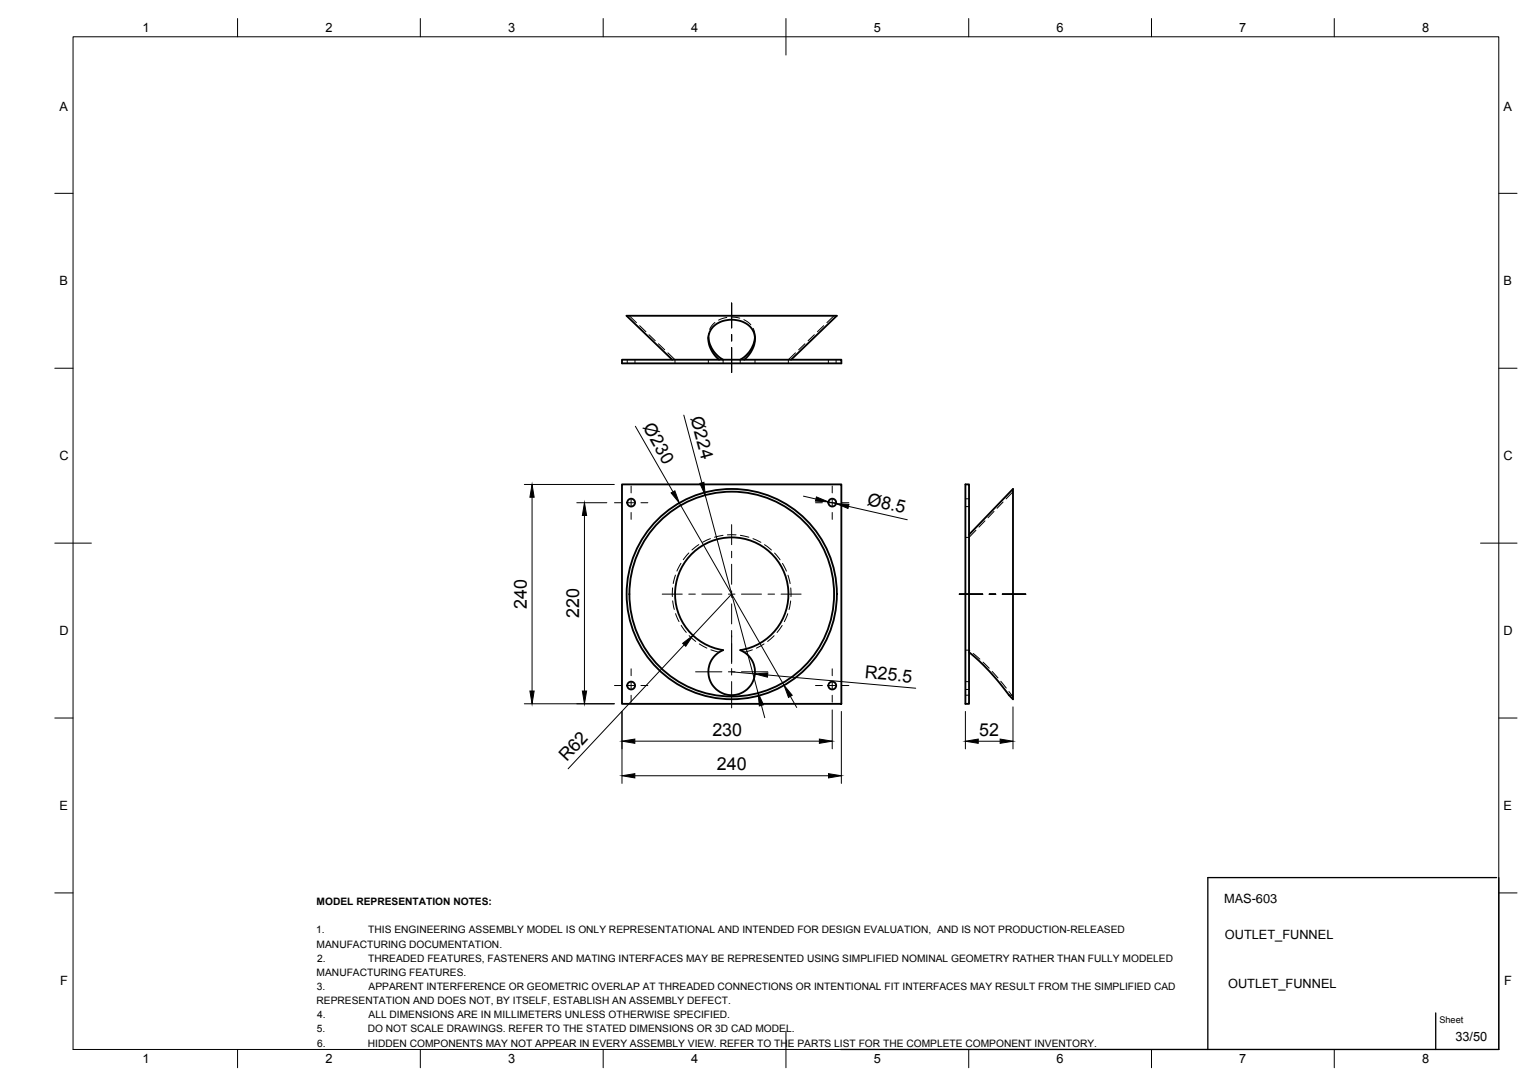
ISO-10303-21;
HEADER;
FILE_DESCRIPTION((''),'2;1');
FILE_NAME('OUTLET_FUNNEL.step','2026-10-01T22:06:14-07:00',(''),(''),'','','');
FILE_SCHEMA (('AUTOMOTIVE_DESIGN { 1 0 10303 214 3 1 1 }'));
ENDSEC;
DATA;
#10=MECHANICAL_DESIGN_GEOMETRIC_PRESENTATION_REPRESENTATION('',(#1005),#50440);
#19=B_SPLINE_CURVE_WITH_KNOTS('',3,(#46833,#46834,#46835,#46836,#46837,
#46838,#46839,#46840,#46841,#46842,#46843,#46844,#46845,#46846,#46847,#46848,
#46849,#46850,#46851,#46852,#46853,#46854,#46855,#46856,#46857,#46858,#46859,
#46860,#46861,#46862,#46863,#46864,#46865,#46866,#46867,#46868,#46869,#46870,
#46871,#46872,#46873,#46874,#46875,#46876,#46877,#46878,#46879),
 .UNSPECIFIED.,.F.,.F.,(4,2,2,2,2,2,2,2,2,2,2,2,2,2,2,2,2,2,2,3,2,2,4),
(-13.6435660379385,-13.1032156835778,-11.9806697877857,-10.8581238919937,
-10.1062638186437,-9.35440374529371,-8.60254367194372,-7.85068359859374,
-7.19512813941189,-6.53957268023004,-5.98431731311344,-5.42906194599684,
-4.87380657888023,-4.31855121176363,-3.66299575258178,-3.00744029339993,
-2.25558022004995,-1.50372014669997,-0.751860073349981,0.,1.12254589579207,
2.24509179158414,2.78544215194592),.UNSPECIFIED.) ;
#20=B_SPLINE_CURVE_WITH_KNOTS('',3,(#46883,#46884,#46885,#46886,#46887,
#46888,#46889,#46890,#46891,#46892,#46893,#46894,#46895,#46896,#46897,#46898,
#46899,#46900,#46901,#46902,#46903,#46904,#46905,#46906,#46907,#46908,#46909,
#46910,#46911,#46912,#46913,#46914,#46915,#46916,#46917,#46918,#46919,#46920,
#46921,#46922,#46923,#46924,#46925),.UNSPECIFIED.,.F.,.F.,(4,2,3,2,2,2,
2,2,2,2,2,2,2,2,2,2,2,2,2,2,4),(-2.23663632321178,-1.12254589579207,0.,
0.751860073349982,1.50372014669996,2.25558022004995,3.00744029339993,3.66299575258178,
4.31855121176363,4.87380657888023,5.42906194599683,5.98431731311343,6.53957268023004,
7.19512813941189,7.85068359859374,8.60254367194372,9.3544037452937,10.1062638186437,
10.8581238919937,11.9806697877857,13.0947602152054),.UNSPECIFIED.) ;
#913=SHAPE_REPRESENTATION_RELATIONSHIP('SRR','None',#50646,#958) ;
#958=ADVANCED_BREP_SHAPE_REPRESENTATION('',(#1060),#50415) ;
#1005=STYLED_ITEM('',(#50889),#1060) ;
#1060=MANIFOLD_SOLID_BREP('OUTLET_FUNNEL',#28672) ;
#1092=CONICAL_SURFACE('',#30829,9.,0.805803494083987) ;
#1093=CONICAL_SURFACE('',#30838,8.7,0.805803494083986) ;
#1338=FACE_BOUND('',#5137,.T.) ;
#1339=FACE_BOUND('',#5139,.T.) ;
#1340=FACE_BOUND('',#5140,.T.) ;
#1341=FACE_BOUND('',#5141,.T.) ;
#1342=FACE_BOUND('',#5142,.T.) ;
#1343=FACE_BOUND('',#5143,.T.) ;
#1344=FACE_BOUND('',#5147,.T.) ;
#1345=FACE_BOUND('',#5148,.T.) ;
#1346=FACE_BOUND('',#5149,.T.) ;
#1347=FACE_BOUND('',#5150,.T.) ;
#1348=FACE_BOUND('',#5151,.T.) ;
#1349=FACE_BOUND('',#5158,.T.) ;
#2194=PLANE('',#30824) ;
#2195=PLANE('',#30833) ;
#2196=PLANE('',#30834) ;
#2197=PLANE('',#30835) ;
#2198=PLANE('',#30836) ;
#2199=PLANE('',#30837) ;
#2200=PLANE('',#30840) ;
#3352=FACE_OUTER_BOUND('',#5132,.T.) ;
#3353=FACE_OUTER_BOUND('',#5133,.T.) ;
#3354=FACE_OUTER_BOUND('',#5134,.T.) ;
#3355=FACE_OUTER_BOUND('',#5135,.T.) ;
#3356=FACE_OUTER_BOUND('',#5136,.T.) ;
#3357=FACE_OUTER_BOUND('',#5138,.T.) ;
#3358=FACE_OUTER_BOUND('',#5144,.T.) ;
#3359=FACE_OUTER_BOUND('',#5145,.T.) ;
#3360=FACE_OUTER_BOUND('',#5146,.T.) ;
#3361=FACE_OUTER_BOUND('',#5152,.T.) ;
#3362=FACE_OUTER_BOUND('',#5153,.T.) ;
#3363=FACE_OUTER_BOUND('',#5154,.T.) ;
#3364=FACE_OUTER_BOUND('',#5155,.T.) ;
#3365=FACE_OUTER_BOUND('',#5156,.T.) ;
#3366=FACE_OUTER_BOUND('',#5157,.T.) ;
#5132=EDGE_LOOP('',(#23817,#23818,#23819,#23820)) ;
#5133=EDGE_LOOP('',(#23821,#23822,#23823,#23824)) ;
#5134=EDGE_LOOP('',(#23825,#23826,#23827,#23828)) ;
#5135=EDGE_LOOP('',(#23829,#23830,#23831,#23832)) ;
#5136=EDGE_LOOP('',(#23833,#23834,#23835,#23836)) ;
#5137=EDGE_LOOP('',(#23837,#23838)) ;
#5138=EDGE_LOOP('',(#23839,#23840,#23841,#23842)) ;
#5139=EDGE_LOOP('',(#23843)) ;
#5140=EDGE_LOOP('',(#23844)) ;
#5141=EDGE_LOOP('',(#23845)) ;
#5142=EDGE_LOOP('',(#23846)) ;
#5143=EDGE_LOOP('',(#23847,#23848)) ;
#5144=EDGE_LOOP('',(#23849,#23850,#23851,#23852,#23853)) ;
#5145=EDGE_LOOP('',(#23854,#23855,#23856,#23857,#23858,#23859)) ;
#5146=EDGE_LOOP('',(#23860,#23861,#23862,#23863)) ;
#5147=EDGE_LOOP('',(#23864)) ;
#5148=EDGE_LOOP('',(#23865)) ;
#5149=EDGE_LOOP('',(#23866)) ;
#5150=EDGE_LOOP('',(#23867)) ;
#5151=EDGE_LOOP('',(#23868,#23869,#23870)) ;
#5152=EDGE_LOOP('',(#23871,#23872,#23873,#23874)) ;
#5153=EDGE_LOOP('',(#23875,#23876,#23877,#23878)) ;
#5154=EDGE_LOOP('',(#23879,#23880,#23881,#23882)) ;
#5155=EDGE_LOOP('',(#23883,#23884,#23885,#23886)) ;
#5156=EDGE_LOOP('',(#23887,#23888,#23889,#23890,#23891,#23892)) ;
#5157=EDGE_LOOP('',(#23893)) ;
#5158=EDGE_LOOP('',(#23894)) ;
#7799=LINE('',#46805,#10271) ;
#7800=LINE('',#46811,#10272) ;
#7801=LINE('',#46817,#10273) ;
#7802=LINE('',#46823,#10274) ;
#7803=LINE('',#46828,#10275) ;
#7804=LINE('',#46832,#10276) ;
#7805=LINE('',#46929,#10277) ;
#7806=LINE('',#46931,#10278) ;
#7807=LINE('',#46933,#10279) ;
#7808=LINE('',#46934,#10280) ;
#7809=LINE('',#46944,#10281) ;
#7810=LINE('',#46950,#10282) ;
#7811=LINE('',#46952,#10283) ;
#7812=LINE('',#46954,#10284) ;
#7813=LINE('',#46955,#10285) ;
#7814=LINE('',#46957,#10286) ;
#7815=LINE('',#46958,#10287) ;
#7816=LINE('',#46960,#10288) ;
#7817=LINE('',#46962,#10289) ;
#7818=LINE('',#46966,#10290) ;
#10271=VECTOR('',#37646,0.425) ;
#10272=VECTOR('',#37653,0.425) ;
#10273=VECTOR('',#37660,0.425) ;
#10274=VECTOR('',#37667,0.425) ;
#10275=VECTOR('',#37672,1.) ;
#10276=VECTOR('',#37675,1.) ;
#10277=VECTOR('',#37680,1.) ;
#10278=VECTOR('',#37681,1.) ;
#10279=VECTOR('',#37682,1.) ;
#10280=VECTOR('',#37683,1.) ;
#10281=VECTOR('',#37696,9.) ;
#10282=VECTOR('',#37703,1.) ;
#10283=VECTOR('',#37704,1.) ;
#10284=VECTOR('',#37705,1.) ;
#10285=VECTOR('',#37706,1.) ;
#10286=VECTOR('',#37709,1.) ;
#10287=VECTOR('',#37710,1.) ;
#10288=VECTOR('',#37713,1.) ;
#10289=VECTOR('',#37716,1.) ;
#10290=VECTOR('',#37721,8.7) ;
#11179=CIRCLE('',#30810,0.425) ;
#11180=CIRCLE('',#30811,0.425) ;
#11181=CIRCLE('',#30813,0.425) ;
#11182=CIRCLE('',#30814,0.425) ;
#11183=CIRCLE('',#30816,0.425) ;
#11184=CIRCLE('',#30817,0.425) ;
#11185=CIRCLE('',#30819,0.425) ;
#11186=CIRCLE('',#30820,0.425) ;
#11187=CIRCLE('',#30822,2.55) ;
#11188=CIRCLE('',#30823,2.55) ;
#11189=CIRCLE('',#30825,6.2) ;
#11190=CIRCLE('',#30827,6.2) ;
#11191=CIRCLE('',#30828,6.2) ;
#11192=CIRCLE('',#30830,11.5) ;
#11193=CIRCLE('',#30831,6.5) ;
#11194=CIRCLE('',#30832,6.5) ;
#11195=CIRCLE('',#30839,11.2) ;
#13588=VERTEX_POINT('',#46802) ;
#13589=VERTEX_POINT('',#46804) ;
#13590=VERTEX_POINT('',#46808) ;
#13591=VERTEX_POINT('',#46810) ;
#13592=VERTEX_POINT('',#46814) ;
#13593=VERTEX_POINT('',#46816) ;
#13594=VERTEX_POINT('',#46820) ;
#13595=VERTEX_POINT('',#46822) ;
#13596=VERTEX_POINT('',#46826) ;
#13597=VERTEX_POINT('',#46827) ;
#13598=VERTEX_POINT('',#46829) ;
#13599=VERTEX_POINT('',#46831) ;
#13600=VERTEX_POINT('',#46880) ;
#13601=VERTEX_POINT('',#46881) ;
#13602=VERTEX_POINT('',#46927) ;
#13603=VERTEX_POINT('',#46928) ;
#13604=VERTEX_POINT('',#46930) ;
#13605=VERTEX_POINT('',#46932) ;
#13606=VERTEX_POINT('',#46937) ;
#13607=VERTEX_POINT('',#46941) ;
#13608=VERTEX_POINT('',#46943) ;
#13609=VERTEX_POINT('',#46948) ;
#13610=VERTEX_POINT('',#46949) ;
#13611=VERTEX_POINT('',#46951) ;
#13612=VERTEX_POINT('',#46953) ;
#13613=VERTEX_POINT('',#46965) ;
#17174=EDGE_CURVE('',#13588,#13588,#11179,.T.) ;
#17175=EDGE_CURVE('',#13588,#13589,#7799,.T.) ;
#17176=EDGE_CURVE('',#13589,#13589,#11180,.T.) ;
#17177=EDGE_CURVE('',#13590,#13590,#11181,.T.) ;
#17178=EDGE_CURVE('',#13590,#13591,#7800,.T.) ;
#17179=EDGE_CURVE('',#13591,#13591,#11182,.T.) ;
#17180=EDGE_CURVE('',#13592,#13592,#11183,.T.) ;
#17181=EDGE_CURVE('',#13592,#13593,#7801,.T.) ;
#17182=EDGE_CURVE('',#13593,#13593,#11184,.T.) ;
#17183=EDGE_CURVE('',#13594,#13594,#11185,.T.) ;
#17184=EDGE_CURVE('',#13594,#13595,#7802,.T.) ;
#17185=EDGE_CURVE('',#13595,#13595,#11186,.T.) ;
#17186=EDGE_CURVE('',#13596,#13597,#7803,.T.) ;
#17187=EDGE_CURVE('',#13598,#13596,#11187,.T.) ;
#17188=EDGE_CURVE('',#13599,#13598,#7804,.T.) ;
#17189=EDGE_CURVE('',#13597,#13599,#19,.T.) ;
#17190=EDGE_CURVE('',#13600,#13601,#11188,.T.) ;
#17191=EDGE_CURVE('',#13601,#13600,#20,.T.) ;
#17192=EDGE_CURVE('',#13602,#13603,#7805,.T.) ;
#17193=EDGE_CURVE('',#13603,#13604,#7806,.T.) ;
#17194=EDGE_CURVE('',#13604,#13605,#7807,.T.) ;
#17195=EDGE_CURVE('',#13605,#13602,#7808,.T.) ;
#17196=EDGE_CURVE('',#13596,#13598,#11189,.T.) ;
#17197=EDGE_CURVE('',#13597,#13606,#11190,.T.) ;
#17198=EDGE_CURVE('',#13606,#13599,#11191,.T.) ;
#17199=EDGE_CURVE('',#13607,#13607,#11192,.T.) ;
#17200=EDGE_CURVE('',#13607,#13608,#7809,.T.) ;
#17201=EDGE_CURVE('',#13601,#13608,#11193,.T.) ;
#17202=EDGE_CURVE('',#13608,#13600,#11194,.T.) ;
#17203=EDGE_CURVE('',#13609,#13610,#7810,.T.) ;
#17204=EDGE_CURVE('',#13610,#13611,#7811,.T.) ;
#17205=EDGE_CURVE('',#13611,#13612,#7812,.T.) ;
#17206=EDGE_CURVE('',#13612,#13609,#7813,.T.) ;
#17207=EDGE_CURVE('',#13612,#13604,#7814,.T.) ;
#17208=EDGE_CURVE('',#13609,#13603,#7815,.T.) ;
#17209=EDGE_CURVE('',#13611,#13605,#7816,.T.) ;
#17210=EDGE_CURVE('',#13610,#13602,#7817,.T.) ;
#17211=EDGE_CURVE('',#13606,#13613,#7818,.T.) ;
#17212=EDGE_CURVE('',#13613,#13613,#11195,.T.) ;
#23817=ORIENTED_EDGE('',*,*,#17174,.F.) ;
#23818=ORIENTED_EDGE('',*,*,#17175,.T.) ;
#23819=ORIENTED_EDGE('',*,*,#17176,.F.) ;
#23820=ORIENTED_EDGE('',*,*,#17175,.F.) ;
#23821=ORIENTED_EDGE('',*,*,#17177,.F.) ;
#23822=ORIENTED_EDGE('',*,*,#17178,.T.) ;
#23823=ORIENTED_EDGE('',*,*,#17179,.F.) ;
#23824=ORIENTED_EDGE('',*,*,#17178,.F.) ;
#23825=ORIENTED_EDGE('',*,*,#17180,.F.) ;
#23826=ORIENTED_EDGE('',*,*,#17181,.T.) ;
#23827=ORIENTED_EDGE('',*,*,#17182,.F.) ;
#23828=ORIENTED_EDGE('',*,*,#17181,.F.) ;
#23829=ORIENTED_EDGE('',*,*,#17183,.F.) ;
#23830=ORIENTED_EDGE('',*,*,#17184,.T.) ;
#23831=ORIENTED_EDGE('',*,*,#17185,.F.) ;
#23832=ORIENTED_EDGE('',*,*,#17184,.F.) ;
#23833=ORIENTED_EDGE('',*,*,#17186,.F.) ;
#23834=ORIENTED_EDGE('',*,*,#17187,.F.) ;
#23835=ORIENTED_EDGE('',*,*,#17188,.F.) ;
#23836=ORIENTED_EDGE('',*,*,#17189,.F.) ;
#23837=ORIENTED_EDGE('',*,*,#17190,.F.) ;
#23838=ORIENTED_EDGE('',*,*,#17191,.F.) ;
#23839=ORIENTED_EDGE('',*,*,#17192,.T.) ;
#23840=ORIENTED_EDGE('',*,*,#17193,.T.) ;
#23841=ORIENTED_EDGE('',*,*,#17194,.T.) ;
#23842=ORIENTED_EDGE('',*,*,#17195,.T.) ;
#23843=ORIENTED_EDGE('',*,*,#17174,.T.) ;
#23844=ORIENTED_EDGE('',*,*,#17177,.T.) ;
#23845=ORIENTED_EDGE('',*,*,#17180,.T.) ;
#23846=ORIENTED_EDGE('',*,*,#17183,.T.) ;
#23847=ORIENTED_EDGE('',*,*,#17187,.T.) ;
#23848=ORIENTED_EDGE('',*,*,#17196,.T.) ;
#23849=ORIENTED_EDGE('',*,*,#17188,.T.) ;
#23850=ORIENTED_EDGE('',*,*,#17196,.F.) ;
#23851=ORIENTED_EDGE('',*,*,#17186,.T.) ;
#23852=ORIENTED_EDGE('',*,*,#17197,.T.) ;
#23853=ORIENTED_EDGE('',*,*,#17198,.T.) ;
#23854=ORIENTED_EDGE('',*,*,#17199,.F.) ;
#23855=ORIENTED_EDGE('',*,*,#17200,.T.) ;
#23856=ORIENTED_EDGE('',*,*,#17201,.F.) ;
#23857=ORIENTED_EDGE('',*,*,#17191,.T.) ;
#23858=ORIENTED_EDGE('',*,*,#17202,.F.) ;
#23859=ORIENTED_EDGE('',*,*,#17200,.F.) ;
#23860=ORIENTED_EDGE('',*,*,#17203,.T.) ;
#23861=ORIENTED_EDGE('',*,*,#17204,.T.) ;
#23862=ORIENTED_EDGE('',*,*,#17205,.T.) ;
#23863=ORIENTED_EDGE('',*,*,#17206,.T.) ;
#23864=ORIENTED_EDGE('',*,*,#17176,.T.) ;
#23865=ORIENTED_EDGE('',*,*,#17179,.T.) ;
#23866=ORIENTED_EDGE('',*,*,#17182,.T.) ;
#23867=ORIENTED_EDGE('',*,*,#17185,.T.) ;
#23868=ORIENTED_EDGE('',*,*,#17190,.T.) ;
#23869=ORIENTED_EDGE('',*,*,#17201,.T.) ;
#23870=ORIENTED_EDGE('',*,*,#17202,.T.) ;
#23871=ORIENTED_EDGE('',*,*,#17207,.T.) ;
#23872=ORIENTED_EDGE('',*,*,#17193,.F.) ;
#23873=ORIENTED_EDGE('',*,*,#17208,.F.) ;
#23874=ORIENTED_EDGE('',*,*,#17206,.F.) ;
#23875=ORIENTED_EDGE('',*,*,#17209,.T.) ;
#23876=ORIENTED_EDGE('',*,*,#17194,.F.) ;
#23877=ORIENTED_EDGE('',*,*,#17207,.F.) ;
#23878=ORIENTED_EDGE('',*,*,#17205,.F.) ;
#23879=ORIENTED_EDGE('',*,*,#17210,.T.) ;
#23880=ORIENTED_EDGE('',*,*,#17195,.F.) ;
#23881=ORIENTED_EDGE('',*,*,#17209,.F.) ;
#23882=ORIENTED_EDGE('',*,*,#17204,.F.) ;
#23883=ORIENTED_EDGE('',*,*,#17208,.T.) ;
#23884=ORIENTED_EDGE('',*,*,#17192,.F.) ;
#23885=ORIENTED_EDGE('',*,*,#17210,.F.) ;
#23886=ORIENTED_EDGE('',*,*,#17203,.F.) ;
#23887=ORIENTED_EDGE('',*,*,#17189,.T.) ;
#23888=ORIENTED_EDGE('',*,*,#17198,.F.) ;
#23889=ORIENTED_EDGE('',*,*,#17211,.T.) ;
#23890=ORIENTED_EDGE('',*,*,#17212,.F.) ;
#23891=ORIENTED_EDGE('',*,*,#17211,.F.) ;
#23892=ORIENTED_EDGE('',*,*,#17197,.F.) ;
#23893=ORIENTED_EDGE('',*,*,#17199,.T.) ;
#23894=ORIENTED_EDGE('',*,*,#17212,.T.) ;
#26847=CYLINDRICAL_SURFACE('',#30809,0.425) ;
#26848=CYLINDRICAL_SURFACE('',#30812,0.425) ;
#26849=CYLINDRICAL_SURFACE('',#30815,0.425) ;
#26850=CYLINDRICAL_SURFACE('',#30818,0.425) ;
#26851=CYLINDRICAL_SURFACE('',#30821,2.55) ;
#26852=CYLINDRICAL_SURFACE('',#30826,6.2) ;
#28087=ADVANCED_FACE('',(#3352),#26847,.F.) ;
#28088=ADVANCED_FACE('',(#3353),#26848,.F.) ;
#28089=ADVANCED_FACE('',(#3354),#26849,.F.) ;
#28090=ADVANCED_FACE('',(#3355),#26850,.F.) ;
#28091=ADVANCED_FACE('',(#3356,#1338),#26851,.F.) ;
#28092=ADVANCED_FACE('',(#3357,#1339,#1340,#1341,#1342,#1343),#2194,.F.) ;
#28093=ADVANCED_FACE('',(#3358),#26852,.F.) ;
#28094=ADVANCED_FACE('',(#3359),#1092,.T.) ;
#28095=ADVANCED_FACE('',(#3360,#1344,#1345,#1346,#1347,#1348),#2195,.T.) ;
#28096=ADVANCED_FACE('',(#3361),#2196,.F.) ;
#28097=ADVANCED_FACE('',(#3362),#2197,.F.) ;
#28098=ADVANCED_FACE('',(#3363),#2198,.F.) ;
#28099=ADVANCED_FACE('',(#3364),#2199,.F.) ;
#28100=ADVANCED_FACE('',(#3365),#1093,.F.) ;
#28101=ADVANCED_FACE('',(#3366,#1349),#2200,.T.) ;
#28672=CLOSED_SHELL('',(#28087,#28088,#28089,#28090,#28091,#28092,#28093,
#28094,#28095,#28096,#28097,#28098,#28099,#28100,#28101)) ;
#30808=AXIS2_PLACEMENT_3D('',#46800,#37640,#37641) ;
#30809=AXIS2_PLACEMENT_3D('',#46801,#37642,#37643) ;
#30810=AXIS2_PLACEMENT_3D('',#46803,#37644,#37645) ;
#30811=AXIS2_PLACEMENT_3D('',#46806,#37647,#37648) ;
#30812=AXIS2_PLACEMENT_3D('',#46807,#37649,#37650) ;
#30813=AXIS2_PLACEMENT_3D('',#46809,#37651,#37652) ;
#30814=AXIS2_PLACEMENT_3D('',#46812,#37654,#37655) ;
#30815=AXIS2_PLACEMENT_3D('',#46813,#37656,#37657) ;
#30816=AXIS2_PLACEMENT_3D('',#46815,#37658,#37659) ;
#30817=AXIS2_PLACEMENT_3D('',#46818,#37661,#37662) ;
#30818=AXIS2_PLACEMENT_3D('',#46819,#37663,#37664) ;
#30819=AXIS2_PLACEMENT_3D('',#46821,#37665,#37666) ;
#30820=AXIS2_PLACEMENT_3D('',#46824,#37668,#37669) ;
#30821=AXIS2_PLACEMENT_3D('',#46825,#37670,#37671) ;
#30822=AXIS2_PLACEMENT_3D('',#46830,#37673,#37674) ;
#30823=AXIS2_PLACEMENT_3D('',#46882,#37676,#37677) ;
#30824=AXIS2_PLACEMENT_3D('',#46926,#37678,#37679) ;
#30825=AXIS2_PLACEMENT_3D('',#46935,#37684,#37685) ;
#30826=AXIS2_PLACEMENT_3D('',#46936,#37686,#37687) ;
#30827=AXIS2_PLACEMENT_3D('',#46938,#37688,#37689) ;
#30828=AXIS2_PLACEMENT_3D('',#46939,#37690,#37691) ;
#30829=AXIS2_PLACEMENT_3D('',#46940,#37692,#37693) ;
#30830=AXIS2_PLACEMENT_3D('',#46942,#37694,#37695) ;
#30831=AXIS2_PLACEMENT_3D('',#46945,#37697,#37698) ;
#30832=AXIS2_PLACEMENT_3D('',#46946,#37699,#37700) ;
#30833=AXIS2_PLACEMENT_3D('',#46947,#37701,#37702) ;
#30834=AXIS2_PLACEMENT_3D('',#46956,#37707,#37708) ;
#30835=AXIS2_PLACEMENT_3D('',#46959,#37711,#37712) ;
#30836=AXIS2_PLACEMENT_3D('',#46961,#37714,#37715) ;
#30837=AXIS2_PLACEMENT_3D('',#46963,#37717,#37718) ;
#30838=AXIS2_PLACEMENT_3D('',#46964,#37719,#37720) ;
#30839=AXIS2_PLACEMENT_3D('',#46967,#37722,#37723) ;
#30840=AXIS2_PLACEMENT_3D('',#46968,#37724,#37725) ;
#37640=DIRECTION('axis',(0.,0.,1.)) ;
#37641=DIRECTION('refdir',(1.,0.,0.)) ;
#37642=DIRECTION('center_axis',(0.,0.,1.)) ;
#37643=DIRECTION('ref_axis',(1.,0.,0.)) ;
#37644=DIRECTION('center_axis',(0.,0.,1.)) ;
#37645=DIRECTION('ref_axis',(1.,0.,0.)) ;
#37646=DIRECTION('',(0.,0.,1.)) ;
#37647=DIRECTION('center_axis',(0.,0.,-1.)) ;
#37648=DIRECTION('ref_axis',(1.,0.,0.)) ;
#37649=DIRECTION('center_axis',(0.,0.,1.)) ;
#37650=DIRECTION('ref_axis',(1.,0.,0.)) ;
#37651=DIRECTION('center_axis',(0.,0.,1.)) ;
#37652=DIRECTION('ref_axis',(1.,0.,0.)) ;
#37653=DIRECTION('',(0.,0.,1.)) ;
#37654=DIRECTION('center_axis',(0.,0.,-1.)) ;
#37655=DIRECTION('ref_axis',(1.,0.,0.)) ;
#37656=DIRECTION('center_axis',(0.,0.,1.)) ;
#37657=DIRECTION('ref_axis',(1.,0.,0.)) ;
#37658=DIRECTION('center_axis',(0.,0.,1.)) ;
#37659=DIRECTION('ref_axis',(1.,0.,0.)) ;
#37660=DIRECTION('',(0.,0.,1.)) ;
#37661=DIRECTION('center_axis',(0.,0.,-1.)) ;
#37662=DIRECTION('ref_axis',(1.,0.,0.)) ;
#37663=DIRECTION('center_axis',(0.,0.,1.)) ;
#37664=DIRECTION('ref_axis',(1.,0.,0.)) ;
#37665=DIRECTION('center_axis',(0.,0.,1.)) ;
#37666=DIRECTION('ref_axis',(1.,0.,0.)) ;
#37667=DIRECTION('',(0.,0.,1.)) ;
#37668=DIRECTION('center_axis',(0.,0.,-1.)) ;
#37669=DIRECTION('ref_axis',(1.,0.,0.)) ;
#37670=DIRECTION('center_axis',(0.,0.,1.)) ;
#37671=DIRECTION('ref_axis',(6.12323399573677E-17,-1.,0.)) ;
#37672=DIRECTION('',(0.,0.,1.)) ;
#37673=DIRECTION('center_axis',(0.,0.,1.)) ;
#37674=DIRECTION('ref_axis',(1.,0.,0.)) ;
#37675=DIRECTION('',(0.,0.,-1.)) ;
#37676=DIRECTION('center_axis',(0.,0.,-1.)) ;
#37677=DIRECTION('ref_axis',(1.,0.,0.)) ;
#37678=DIRECTION('center_axis',(0.,0.,1.)) ;
#37679=DIRECTION('ref_axis',(1.,0.,0.)) ;
#37680=DIRECTION('',(0.,-1.,0.)) ;
#37681=DIRECTION('',(-1.,0.,0.)) ;
#37682=DIRECTION('',(0.,1.,0.)) ;
#37683=DIRECTION('',(1.,0.,0.)) ;
#37684=DIRECTION('center_axis',(0.,0.,1.)) ;
#37685=DIRECTION('ref_axis',(1.,0.,0.)) ;
#37686=DIRECTION('center_axis',(0.,0.,1.)) ;
#37687=DIRECTION('ref_axis',(-1.83697019872103E-16,1.,0.)) ;
#37688=DIRECTION('center_axis',(0.,0.,1.)) ;
#37689=DIRECTION('ref_axis',(1.,0.,0.)) ;
#37690=DIRECTION('center_axis',(0.,0.,1.)) ;
#37691=DIRECTION('ref_axis',(1.,0.,0.)) ;
#37692=DIRECTION('center_axis',(0.,0.,1.)) ;
#37693=DIRECTION('ref_axis',(1.,0.,0.)) ;
#37694=DIRECTION('center_axis',(0.,0.,1.)) ;
#37695=DIRECTION('ref_axis',(1.,0.,0.)) ;
#37696=DIRECTION('',(0.721387321030952,8.83444673646039E-17,-0.692531828189713)) ;
#37697=DIRECTION('center_axis',(0.,0.,-1.)) ;
#37698=DIRECTION('ref_axis',(1.,0.,0.)) ;
#37699=DIRECTION('center_axis',(0.,0.,-1.)) ;
#37700=DIRECTION('ref_axis',(1.,0.,0.)) ;
#37701=DIRECTION('center_axis',(0.,0.,1.)) ;
#37702=DIRECTION('ref_axis',(1.,0.,0.)) ;
#37703=DIRECTION('',(0.,1.,0.)) ;
#37704=DIRECTION('',(-1.,0.,0.)) ;
#37705=DIRECTION('',(0.,-1.,0.)) ;
#37706=DIRECTION('',(1.,0.,0.)) ;
#37707=DIRECTION('center_axis',(0.,1.,0.)) ;
#37708=DIRECTION('ref_axis',(0.,0.,1.)) ;
#37709=DIRECTION('',(0.,0.,-1.)) ;
#37710=DIRECTION('',(0.,0.,-1.)) ;
#37711=DIRECTION('center_axis',(1.,0.,0.)) ;
#37712=DIRECTION('ref_axis',(0.,0.,-1.)) ;
#37713=DIRECTION('',(0.,0.,-1.)) ;
#37714=DIRECTION('center_axis',(0.,-1.,0.)) ;
#37715=DIRECTION('ref_axis',(0.,0.,-1.)) ;
#37716=DIRECTION('',(0.,0.,-1.)) ;
#37717=DIRECTION('center_axis',(-1.,0.,0.)) ;
#37718=DIRECTION('ref_axis',(0.,0.,1.)) ;
#37719=DIRECTION('center_axis',(0.,0.,1.)) ;
#37720=DIRECTION('ref_axis',(1.,0.,0.)) ;
#37721=DIRECTION('',(-0.721387321030951,-8.83444673646039E-17,0.692531828189713)) ;
#37722=DIRECTION('center_axis',(0.,0.,-1.)) ;
#37723=DIRECTION('ref_axis',(1.,0.,0.)) ;
#37724=DIRECTION('center_axis',(0.,0.,1.)) ;
#37725=DIRECTION('ref_axis',(1.,0.,0.)) ;
#46800=CARTESIAN_POINT('',(0.,0.,0.)) ;
#46801=CARTESIAN_POINT('Origin',(-11.,-10.,43.)) ;
#46802=CARTESIAN_POINT('',(-11.425,-10.,42.8)) ;
#46803=CARTESIAN_POINT('Origin',(-11.,-10.,42.8)) ;
#46804=CARTESIAN_POINT('',(-11.425,-10.,43.2)) ;
#46805=CARTESIAN_POINT('',(-11.425,-10.,43.)) ;
#46806=CARTESIAN_POINT('Origin',(-11.,-10.,43.2)) ;
#46807=CARTESIAN_POINT('Origin',(-11.,10.,43.)) ;
#46808=CARTESIAN_POINT('',(-11.425,10.,42.8)) ;
#46809=CARTESIAN_POINT('Origin',(-11.,10.,42.8)) ;
#46810=CARTESIAN_POINT('',(-11.425,10.,43.2)) ;
#46811=CARTESIAN_POINT('',(-11.425,10.,43.)) ;
#46812=CARTESIAN_POINT('Origin',(-11.,10.,43.2)) ;
#46813=CARTESIAN_POINT('Origin',(11.,-10.,43.)) ;
#46814=CARTESIAN_POINT('',(10.575,-10.,42.8)) ;
#46815=CARTESIAN_POINT('Origin',(11.,-10.,42.8)) ;
#46816=CARTESIAN_POINT('',(10.575,-10.,43.2)) ;
#46817=CARTESIAN_POINT('',(10.575,-10.,43.)) ;
#46818=CARTESIAN_POINT('Origin',(11.,-10.,43.2)) ;
#46819=CARTESIAN_POINT('Origin',(11.,10.,43.)) ;
#46820=CARTESIAN_POINT('',(10.575,10.,42.8)) ;
#46821=CARTESIAN_POINT('Origin',(11.,10.,42.8)) ;
#46822=CARTESIAN_POINT('',(10.575,10.,43.2)) ;
#46823=CARTESIAN_POINT('',(10.575,10.,43.)) ;
#46824=CARTESIAN_POINT('Origin',(11.,10.,43.2)) ;
#46825=CARTESIAN_POINT('Origin',(0.,-8.5,45.4)) ;
#46826=CARTESIAN_POINT('',(0.937723156831554,-6.12867647058824,42.8)) ;
#46827=CARTESIAN_POINT('',(0.937723156831558,-6.12867647058824,43.2)) ;
#46828=CARTESIAN_POINT('',(0.937723156831553,-6.12867647058824,45.4)) ;
#46829=CARTESIAN_POINT('',(-0.937723156831554,-6.12867647058824,42.8)) ;
#46830=CARTESIAN_POINT('Origin',(0.,-8.5,42.8)) ;
#46831=CARTESIAN_POINT('',(-0.937723156831558,-6.12867647058824,43.2)) ;
#46832=CARTESIAN_POINT('',(-0.937723156831553,-6.12867647058824,45.4)) ;
#46833=CARTESIAN_POINT('Ctrl Pts',(0.937723156831556,-6.12867647058824,
43.2)) ;
#46834=CARTESIAN_POINT('Ctrl Pts',(1.09784051872832,-6.19199375150714,43.283333711661)) ;
#46835=CARTESIAN_POINT('Ctrl Pts',(1.24365353256702,-6.26883036968412,43.3825149112026)) ;
#46836=CARTESIAN_POINT('Ctrl Pts',(1.63123265264399,-6.51561417883593,43.692558910546)) ;
#46837=CARTESIAN_POINT('Ctrl Pts',(1.86026484716295,-6.73020299859327,43.9504989662474)) ;
#46838=CARTESIAN_POINT('Ctrl Pts',(2.22065273073428,-7.21102082090391,44.4906901557995)) ;
#46839=CARTESIAN_POINT('Ctrl Pts',(2.35156592596324,-7.47750307164224,44.7730109630824)) ;
#46840=CARTESIAN_POINT('Ctrl Pts',(2.48678319602362,-7.9074665870395,45.2057062272756)) ;
#46841=CARTESIAN_POINT('Ctrl Pts',(2.52462680466552,-8.09269952236317,45.3861655557954)) ;
#46842=CARTESIAN_POINT('Ctrl Pts',(2.55716495223486,-8.476728138187,45.7477877464213)) ;
#46843=CARTESIAN_POINT('Ctrl Pts',(2.5518683936729,-8.67551622138784,45.9289578753981)) ;
#46844=CARTESIAN_POINT('Ctrl Pts',(2.4929255543873,-9.07285134981918,46.2803948513796)) ;
#46845=CARTESIAN_POINT('Ctrl Pts',(2.43925028674063,-9.27156833359866,46.4508409483682)) ;
#46846=CARTESIAN_POINT('Ctrl Pts',(2.28306121904059,-9.65450903825491,46.7712289756871)) ;
#46847=CARTESIAN_POINT('Ctrl Pts',(2.1805386953413,-9.83871335384025,46.9211898465972)) ;
#46848=CARTESIAN_POINT('Ctrl Pts',(1.94718064660289,-10.1567267690656,47.1751631349221)) ;
#46849=CARTESIAN_POINT('Ctrl Pts',(1.80829195391443,-10.3103948601966,47.2955507638619)) ;
#46850=CARTESIAN_POINT('Ctrl Pts',(1.48448994480638,-10.5841638269278,47.5067752387865)) ;
#46851=CARTESIAN_POINT('Ctrl Pts',(1.29928018215051,-10.7039696130829,47.5975398933414)) ;
#46852=CARTESIAN_POINT('Ctrl Pts',(0.954201226528961,-10.8712714438875,
47.7233432510296)) ;
#46853=CARTESIAN_POINT('Ctrl Pts',(0.770006896249385,-10.9389661797779,
47.7737387327547)) ;
#46854=CARTESIAN_POINT('Ctrl Pts',(0.38547380902765,-11.0284138479361,47.8400994317072)) ;
#46855=CARTESIAN_POINT('Ctrl Pts',(0.1850851223722,-11.05,47.856)) ;
#46856=CARTESIAN_POINT('Ctrl Pts',(-0.1850851223722,-11.05,47.856)) ;
#46857=CARTESIAN_POINT('Ctrl Pts',(-0.38547380902765,-11.0284138479361,
47.8400994317072)) ;
#46858=CARTESIAN_POINT('Ctrl Pts',(-0.770006896249385,-10.9389661797779,
47.7737387327547)) ;
#46859=CARTESIAN_POINT('Ctrl Pts',(-0.954201226528961,-10.8712714438875,
47.7233432510296)) ;
#46860=CARTESIAN_POINT('Ctrl Pts',(-1.29928018215051,-10.7039696130829,
47.5975398933414)) ;
#46861=CARTESIAN_POINT('Ctrl Pts',(-1.48448994480638,-10.5841638269278,
47.5067752387865)) ;
#46862=CARTESIAN_POINT('Ctrl Pts',(-1.80829195391443,-10.3103948601966,
47.2955507638619)) ;
#46863=CARTESIAN_POINT('Ctrl Pts',(-1.94718064660289,-10.1567267690656,
47.1751631349221)) ;
#46864=CARTESIAN_POINT('Ctrl Pts',(-2.1805386953413,-9.83871335384025,46.9211898465972)) ;
#46865=CARTESIAN_POINT('Ctrl Pts',(-2.28306121904059,-9.65450903825491,
46.7712289756871)) ;
#46866=CARTESIAN_POINT('Ctrl Pts',(-2.43925028674063,-9.27156833359864,
46.4508409483682)) ;
#46867=CARTESIAN_POINT('Ctrl Pts',(-2.4929255543873,-9.07285134981916,46.2803948513796)) ;
#46868=CARTESIAN_POINT('Ctrl Pts',(-2.5518683936729,-8.67551622138783,45.9289578753981)) ;
#46869=CARTESIAN_POINT('Ctrl Pts',(-2.55716495223486,-8.47672813818699,
45.7477877464213)) ;
#46870=CARTESIAN_POINT('Ctrl Pts',(-2.52462680466552,-8.09269952236317,
45.3861655557954)) ;
#46871=CARTESIAN_POINT('Ctrl Pts',(-2.48678319602362,-7.9074665870395,45.2057062272756)) ;
#46872=CARTESIAN_POINT('Ctrl Pts',(-2.43254496361321,-7.735,45.0321438835623)) ;
#46873=CARTESIAN_POINT('Ctrl Pts',(-2.35156592596324,-7.47750307164224,
44.7730109630824)) ;
#46874=CARTESIAN_POINT('Ctrl Pts',(-2.22065273073428,-7.21102082090391,
44.4906901557995)) ;
#46875=CARTESIAN_POINT('Ctrl Pts',(-1.86026484716295,-6.73020299859328,
43.9504989662474)) ;
#46876=CARTESIAN_POINT('Ctrl Pts',(-1.63123265264399,-6.51561417883593,
43.692558910546)) ;
#46877=CARTESIAN_POINT('Ctrl Pts',(-1.24365353116831,-6.26883036879351,
43.3825149100837)) ;
#46878=CARTESIAN_POINT('Ctrl Pts',(-1.0978405215343,-6.19199375261675,43.2833337131214)) ;
#46879=CARTESIAN_POINT('Ctrl Pts',(-0.937723156831557,-6.12867647058824,
43.2)) ;
#46880=CARTESIAN_POINT('',(1.37550241686044,-6.35279411764706,43.2)) ;
#46881=CARTESIAN_POINT('',(-1.37550241686044,-6.35279411764706,43.2)) ;
#46882=CARTESIAN_POINT('Origin',(0.,-8.5,43.2)) ;
#46883=CARTESIAN_POINT('Ctrl Pts',(-1.37550241686045,-6.35279411764706,
43.2)) ;
#46884=CARTESIAN_POINT('Ctrl Pts',(-1.63469354395804,-6.51883223475618,
43.4084416977862)) ;
#46885=CARTESIAN_POINT('Ctrl Pts',(-1.86162214059867,-6.73201385546098,
43.6645334351878)) ;
#46886=CARTESIAN_POINT('Ctrl Pts',(-2.22065273073428,-7.21102082090391,
44.2026901557995)) ;
#46887=CARTESIAN_POINT('Ctrl Pts',(-2.35156592596324,-7.47750307164224,
44.4850109630824)) ;
#46888=CARTESIAN_POINT('Ctrl Pts',(-2.43254496361321,-7.735,44.7441438835623)) ;
#46889=CARTESIAN_POINT('Ctrl Pts',(-2.48678319602362,-7.9074665870395,44.9177062272756)) ;
#46890=CARTESIAN_POINT('Ctrl Pts',(-2.52462680466552,-8.09269952236319,
45.0981655557954)) ;
#46891=CARTESIAN_POINT('Ctrl Pts',(-2.55716495223486,-8.47672813818701,
45.4597877464213)) ;
#46892=CARTESIAN_POINT('Ctrl Pts',(-2.5518683936729,-8.67551622138784,45.6409578753981)) ;
#46893=CARTESIAN_POINT('Ctrl Pts',(-2.4929255543873,-9.07285134981917,45.9923948513796)) ;
#46894=CARTESIAN_POINT('Ctrl Pts',(-2.43925028674063,-9.27156833359865,
46.1628409483682)) ;
#46895=CARTESIAN_POINT('Ctrl Pts',(-2.28306121904059,-9.65450903825491,
46.4832289756871)) ;
#46896=CARTESIAN_POINT('Ctrl Pts',(-2.1805386953413,-9.83871335384025,46.6331898465971)) ;
#46897=CARTESIAN_POINT('Ctrl Pts',(-1.94718064660289,-10.1567267690656,
46.8871631349221)) ;
#46898=CARTESIAN_POINT('Ctrl Pts',(-1.80829195391443,-10.3103948601966,
47.0075507638619)) ;
#46899=CARTESIAN_POINT('Ctrl Pts',(-1.48448994480638,-10.5841638269278,
47.2187752387865)) ;
#46900=CARTESIAN_POINT('Ctrl Pts',(-1.29928018215051,-10.7039696130829,
47.3095398933415)) ;
#46901=CARTESIAN_POINT('Ctrl Pts',(-0.954201226528961,-10.8712714438875,
47.4353432510296)) ;
#46902=CARTESIAN_POINT('Ctrl Pts',(-0.770006896249383,-10.9389661797779,
47.4857387327547)) ;
#46903=CARTESIAN_POINT('Ctrl Pts',(-0.385473809027648,-11.0284138479361,
47.5520994317072)) ;
#46904=CARTESIAN_POINT('Ctrl Pts',(-0.185085122372201,-11.05,47.568)) ;
#46905=CARTESIAN_POINT('Ctrl Pts',(0.1850851223722,-11.05,47.568)) ;
#46906=CARTESIAN_POINT('Ctrl Pts',(0.385473809027648,-11.0284138479361,
47.5520994317072)) ;
#46907=CARTESIAN_POINT('Ctrl Pts',(0.770006896249383,-10.9389661797779,
47.4857387327547)) ;
#46908=CARTESIAN_POINT('Ctrl Pts',(0.95420122652896,-10.8712714438875,47.4353432510296)) ;
#46909=CARTESIAN_POINT('Ctrl Pts',(1.29928018215051,-10.7039696130829,47.3095398933415)) ;
#46910=CARTESIAN_POINT('Ctrl Pts',(1.48448994480638,-10.5841638269278,47.2187752387865)) ;
#46911=CARTESIAN_POINT('Ctrl Pts',(1.80829195391443,-10.3103948601966,47.0075507638619)) ;
#46912=CARTESIAN_POINT('Ctrl Pts',(1.94718064660289,-10.1567267690656,46.8871631349221)) ;
#46913=CARTESIAN_POINT('Ctrl Pts',(2.1805386953413,-9.83871335384025,46.6331898465971)) ;
#46914=CARTESIAN_POINT('Ctrl Pts',(2.28306121904059,-9.6545090382549,46.4832289756871)) ;
#46915=CARTESIAN_POINT('Ctrl Pts',(2.43925028674063,-9.27156833359865,46.1628409483682)) ;
#46916=CARTESIAN_POINT('Ctrl Pts',(2.4929255543873,-9.07285134981917,45.9923948513796)) ;
#46917=CARTESIAN_POINT('Ctrl Pts',(2.5518683936729,-8.67551622138783,45.6409578753981)) ;
#46918=CARTESIAN_POINT('Ctrl Pts',(2.55716495223486,-8.47672813818701,45.4597877464213)) ;
#46919=CARTESIAN_POINT('Ctrl Pts',(2.52462680466552,-8.09269952236319,45.0981655557954)) ;
#46920=CARTESIAN_POINT('Ctrl Pts',(2.48678319602362,-7.9074665870395,44.9177062272756)) ;
#46921=CARTESIAN_POINT('Ctrl Pts',(2.35156592596324,-7.47750307164224,44.4850109630824)) ;
#46922=CARTESIAN_POINT('Ctrl Pts',(2.22065273073428,-7.21102082090391,44.2026901557995)) ;
#46923=CARTESIAN_POINT('Ctrl Pts',(1.86162214059868,-6.73201385546098,43.6645334351878)) ;
#46924=CARTESIAN_POINT('Ctrl Pts',(1.63469354395804,-6.51883223475618,43.4084416977862)) ;
#46925=CARTESIAN_POINT('Ctrl Pts',(1.37550241686045,-6.35279411764706,43.2)) ;
#46926=CARTESIAN_POINT('Origin',(0.,0.,42.8)) ;
#46927=CARTESIAN_POINT('',(12.,12.,42.8)) ;
#46928=CARTESIAN_POINT('',(12.,-12.,42.8)) ;
#46929=CARTESIAN_POINT('',(12.,0.,42.8)) ;
#46930=CARTESIAN_POINT('',(-12.,-12.,42.8)) ;
#46931=CARTESIAN_POINT('',(0.,-12.,42.8)) ;
#46932=CARTESIAN_POINT('',(-12.,12.,42.8)) ;
#46933=CARTESIAN_POINT('',(-12.,0.,42.8)) ;
#46934=CARTESIAN_POINT('',(0.,12.,42.8)) ;
#46935=CARTESIAN_POINT('Origin',(0.,0.,42.8)) ;
#46936=CARTESIAN_POINT('Origin',(0.,0.,43.)) ;
#46937=CARTESIAN_POINT('',(-6.2,-7.59281015471359E-16,43.2)) ;
#46938=CARTESIAN_POINT('Origin',(0.,0.,43.2)) ;
#46939=CARTESIAN_POINT('Origin',(0.,0.,43.2)) ;
#46940=CARTESIAN_POINT('Origin',(0.,0.,45.6)) ;
#46941=CARTESIAN_POINT('',(-11.5,-1.40834381901946E-15,48.)) ;
#46942=CARTESIAN_POINT('Origin',(0.,0.,48.)) ;
#46943=CARTESIAN_POINT('',(-6.5,-7.9602041944578E-16,43.2)) ;
#46944=CARTESIAN_POINT('',(-9.,-1.10218211923262E-15,45.6)) ;
#46945=CARTESIAN_POINT('Origin',(0.,0.,43.2)) ;
#46946=CARTESIAN_POINT('Origin',(0.,0.,43.2)) ;
#46947=CARTESIAN_POINT('Origin',(0.,0.,43.2)) ;
#46948=CARTESIAN_POINT('',(12.,-12.,43.2)) ;
#46949=CARTESIAN_POINT('',(12.,12.,43.2)) ;
#46950=CARTESIAN_POINT('',(12.,0.,43.2)) ;
#46951=CARTESIAN_POINT('',(-12.,12.,43.2)) ;
#46952=CARTESIAN_POINT('',(0.,12.,43.2)) ;
#46953=CARTESIAN_POINT('',(-12.,-12.,43.2)) ;
#46954=CARTESIAN_POINT('',(-12.,0.,43.2)) ;
#46955=CARTESIAN_POINT('',(0.,-12.,43.2)) ;
#46956=CARTESIAN_POINT('Origin',(0.,-12.,43.)) ;
#46957=CARTESIAN_POINT('',(-12.,-12.,43.)) ;
#46958=CARTESIAN_POINT('',(12.,-12.,43.)) ;
#46959=CARTESIAN_POINT('Origin',(-12.,0.,43.)) ;
#46960=CARTESIAN_POINT('',(-12.,12.,43.)) ;
#46961=CARTESIAN_POINT('Origin',(0.,12.,43.)) ;
#46962=CARTESIAN_POINT('',(12.,12.,43.)) ;
#46963=CARTESIAN_POINT('Origin',(12.,0.,43.)) ;
#46964=CARTESIAN_POINT('Origin',(0.,0.,45.6)) ;
#46965=CARTESIAN_POINT('',(-11.2,1.37160441504504E-15,48.)) ;
#46966=CARTESIAN_POINT('',(-8.7,-1.0654427152582E-15,45.6)) ;
#46967=CARTESIAN_POINT('Origin',(0.,0.,48.)) ;
#46968=CARTESIAN_POINT('Origin',(0.,0.,48.)) ;
#50362=UNCERTAINTY_MEASURE_WITH_UNIT(LENGTH_MEASURE(0.001),#50441,
'DISTANCE_ACCURACY_VALUE',
'Maximum model space distance between geometric entities at asserted c
onnectivities') ;
#50387=UNCERTAINTY_MEASURE_WITH_UNIT(LENGTH_MEASURE(0.001),#50441,
'DISTANCE_ACCURACY_VALUE',
'Maximum model space distance between geometric entities at asserted c
onnectivities') ;
#50415=(
GEOMETRIC_REPRESENTATION_CONTEXT(3)
GLOBAL_UNCERTAINTY_ASSIGNED_CONTEXT((#50362))
GLOBAL_UNIT_ASSIGNED_CONTEXT((#50441,#50443,#50444))
REPRESENTATION_CONTEXT('','3D')
) ;
#50440=(
GEOMETRIC_REPRESENTATION_CONTEXT(3)
GLOBAL_UNCERTAINTY_ASSIGNED_CONTEXT((#50387))
GLOBAL_UNIT_ASSIGNED_CONTEXT((#50441,#50443,#50444))
REPRESENTATION_CONTEXT('','3D')
) ;
#50441=(
LENGTH_UNIT()
NAMED_UNIT(*)
SI_UNIT(.CENTI.,.METRE.)
) ;
#50443=(
NAMED_UNIT(*)
PLANE_ANGLE_UNIT()
SI_UNIT($,.RADIAN.)
) ;
#50444=(
NAMED_UNIT(*)
SI_UNIT($,.STERADIAN.)
SOLID_ANGLE_UNIT()
) ;
#50472=SHAPE_DEFINITION_REPRESENTATION(#50548,#50646) ;
#50548=PRODUCT_DEFINITION_SHAPE('',$,#50699) ;
#50646=SHAPE_REPRESENTATION('',(#30808),#50415) ;
#50671=PRODUCT_DEFINITION_CONTEXT('part definition',#50829,'design') ;
#50699=PRODUCT_DEFINITION('OUTLET_FUNNEL','OUTLET_FUNNEL',#50751,
#50671) ;
#50751=PRODUCT_DEFINITION_FORMATION('',$,#50858) ;
#50829=APPLICATION_CONTEXT(
'Core Data for Automotive Mechanical Design Process') ;
#50830=PRODUCT_CONTEXT('part definition',#50829,'mechanical') ;
#50858=PRODUCT('OUTLET_FUNNEL','OUTLET_FUNNEL',$,(#50830)) ;
#50889=PRESENTATION_STYLE_ASSIGNMENT((#50896)) ;
#50896=SURFACE_STYLE_USAGE(.BOTH.,#50903) ;
#50903=SURFACE_SIDE_STYLE('',(#50910)) ;
#50910=SURFACE_STYLE_FILL_AREA(#50917) ;
#50917=FILL_AREA_STYLE('Stainless Steel - Satin',(#50924)) ;
#50924=FILL_AREA_STYLE_COLOUR('Stainless Steel - Satin',#50931) ;
#50931=COLOUR_RGB('Stainless Steel - Satin', 0.72549020, 0.75294118, 0.79215686) ;
ENDSEC;
END-ISO-10303-21;
